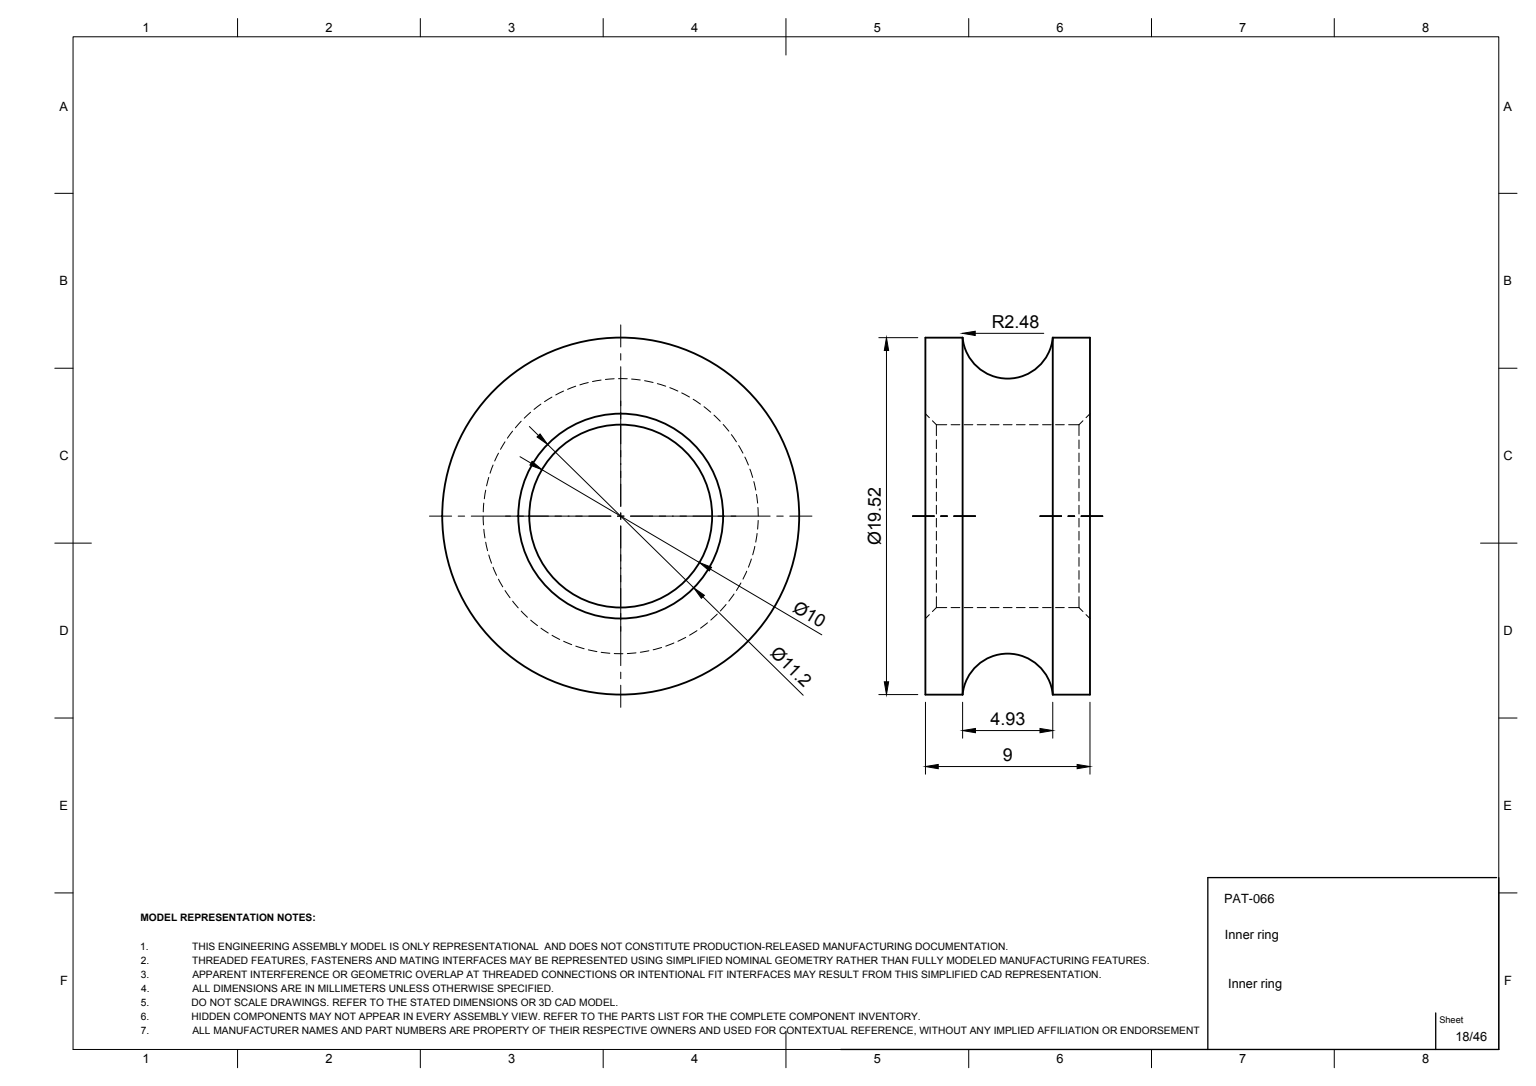
ISO-10303-21;
HEADER;
/* Generated by software containing ST-Developer
 * from STEP Tools, Inc. (www.steptools.com) 
 */

FILE_DESCRIPTION(
/* description */ ('Lever-operated bar clamp (toggle)'),
/* implementation_level */ '2;1');

FILE_NAME(
/* name */ 'Inner ring.step',
/* time_stamp */ '2026-10-28T03:25:02-07:00',
/* author */ (''),
/* organization */ (''),
/* preprocessor_version */ 'ST-DEVELOPER v20.2',
/* originating_system */ 'Autodesk Translation Framework v15.17.0.0',
/* authorisation */ '');

FILE_SCHEMA (('AUTOMOTIVE_DESIGN { 1 0 10303 214 3 1 1 }'));
ENDSEC;

DATA;
#10=MECHANICAL_DESIGN_GEOMETRIC_PRESENTATION_REPRESENTATION('',(#422),#12413);
#303=TOROIDAL_SURFACE('',#7329,1.,0.247676);
#308=CONICAL_SURFACE('',#7340,0.53,0.785398163397448);
#309=CONICAL_SURFACE('',#7347,0.53,0.785398163397448);
#346=SHAPE_REPRESENTATION_RELATIONSHIP('SRR','None',#12586,#384);
#384=ADVANCED_BREP_SHAPE_REPRESENTATION('',(#468),#12383);
#422=STYLED_ITEM('',(#12869),#468);
#468=MANIFOLD_SOLID_BREP('Body1',#6582);
#588=FACE_BOUND('',#1538,.T.);
#589=FACE_BOUND('',#1541,.T.);
#739=PLANE('',#7342);
#740=PLANE('',#7345);
#1039=FACE_OUTER_BOUND('',#1533,.T.);
#1040=FACE_OUTER_BOUND('',#1534,.T.);
#1041=FACE_OUTER_BOUND('',#1535,.T.);
#1042=FACE_OUTER_BOUND('',#1536,.T.);
#1043=FACE_OUTER_BOUND('',#1537,.T.);
#1044=FACE_OUTER_BOUND('',#1539,.T.);
#1045=FACE_OUTER_BOUND('',#1540,.T.);
#1046=FACE_OUTER_BOUND('',#1542,.T.);
#1533=EDGE_LOOP('',(#5045,#5046,#5047,#5048,#5049,#5050));
#1534=EDGE_LOOP('',(#5051,#5052,#5053,#5054,#5055));
#1535=EDGE_LOOP('',(#5056,#5057,#5058,#5059));
#1536=EDGE_LOOP('',(#5060,#5061,#5062,#5063));
#1537=EDGE_LOOP('',(#5064));
#1538=EDGE_LOOP('',(#5065));
#1539=EDGE_LOOP('',(#5066,#5067,#5068,#5069,#5070));
#1540=EDGE_LOOP('',(#5071));
#1541=EDGE_LOOP('',(#5072));
#1542=EDGE_LOOP('',(#5073,#5074,#5075,#5076));
#2040=LINE('',#10743,#2481);
#2041=LINE('',#10749,#2482);
#2042=LINE('',#10753,#2483);
#2043=LINE('',#10759,#2484);
#2044=LINE('',#10764,#2485);
#2481=VECTOR('',#8677,0.976185);
#2482=VECTOR('',#8684,0.5);
#2483=VECTOR('',#8689,0.53);
#2484=VECTOR('',#8698,0.976185);
#2485=VECTOR('',#8705,0.53);
#2856=CIRCLE('',#7330,0.976185);
#2857=CIRCLE('',#7331,0.976185);
#2858=CIRCLE('',#7332,0.247676);
#2859=CIRCLE('',#7333,0.976185);
#2860=CIRCLE('',#7334,0.976185);
#2861=CIRCLE('',#7336,0.976185);
#2862=CIRCLE('',#7338,0.5);
#2863=CIRCLE('',#7339,0.5);
#2864=CIRCLE('',#7341,0.56);
#2865=CIRCLE('',#7344,0.976185);
#2866=CIRCLE('',#7346,0.56);
#3281=VERTEX_POINT('',#10732);
#3282=VERTEX_POINT('',#10733);
#3283=VERTEX_POINT('',#10736);
#3284=VERTEX_POINT('',#10738);
#3285=VERTEX_POINT('',#10742);
#3286=VERTEX_POINT('',#10746);
#3287=VERTEX_POINT('',#10748);
#3288=VERTEX_POINT('',#10752);
#3289=VERTEX_POINT('',#10757);
#3290=VERTEX_POINT('',#10761);
#3927=EDGE_CURVE('',#3281,#3282,#2856,.T.);
#3928=EDGE_CURVE('',#3282,#3281,#2857,.T.);
#3929=EDGE_CURVE('',#3282,#3283,#2858,.T.);
#3930=EDGE_CURVE('',#3284,#3283,#2859,.T.);
#3931=EDGE_CURVE('',#3283,#3284,#2860,.T.);
#3932=EDGE_CURVE('',#3284,#3285,#2040,.T.);
#3933=EDGE_CURVE('',#3285,#3285,#2861,.T.);
#3934=EDGE_CURVE('',#3286,#3286,#2862,.T.);
#3935=EDGE_CURVE('',#3286,#3287,#2041,.T.);
#3936=EDGE_CURVE('',#3287,#3287,#2863,.T.);
#3937=EDGE_CURVE('',#3287,#3288,#2042,.T.);
#3938=EDGE_CURVE('',#3288,#3288,#2864,.T.);
#3939=EDGE_CURVE('',#3289,#3289,#2865,.T.);
#3940=EDGE_CURVE('',#3289,#3281,#2043,.T.);
#3941=EDGE_CURVE('',#3290,#3290,#2866,.T.);
#3942=EDGE_CURVE('',#3290,#3286,#2044,.T.);
#5045=ORIENTED_EDGE('',*,*,#3927,.F.);
#5046=ORIENTED_EDGE('',*,*,#3928,.F.);
#5047=ORIENTED_EDGE('',*,*,#3929,.T.);
#5048=ORIENTED_EDGE('',*,*,#3930,.F.);
#5049=ORIENTED_EDGE('',*,*,#3931,.F.);
#5050=ORIENTED_EDGE('',*,*,#3929,.F.);
#5051=ORIENTED_EDGE('',*,*,#3930,.T.);
#5052=ORIENTED_EDGE('',*,*,#3931,.T.);
#5053=ORIENTED_EDGE('',*,*,#3932,.T.);
#5054=ORIENTED_EDGE('',*,*,#3933,.T.);
#5055=ORIENTED_EDGE('',*,*,#3932,.F.);
#5056=ORIENTED_EDGE('',*,*,#3934,.T.);
#5057=ORIENTED_EDGE('',*,*,#3935,.T.);
#5058=ORIENTED_EDGE('',*,*,#3936,.F.);
#5059=ORIENTED_EDGE('',*,*,#3935,.F.);
#5060=ORIENTED_EDGE('',*,*,#3936,.T.);
#5061=ORIENTED_EDGE('',*,*,#3937,.T.);
#5062=ORIENTED_EDGE('',*,*,#3938,.F.);
#5063=ORIENTED_EDGE('',*,*,#3937,.F.);
#5064=ORIENTED_EDGE('',*,*,#3933,.F.);
#5065=ORIENTED_EDGE('',*,*,#3938,.T.);
#5066=ORIENTED_EDGE('',*,*,#3939,.F.);
#5067=ORIENTED_EDGE('',*,*,#3940,.T.);
#5068=ORIENTED_EDGE('',*,*,#3927,.T.);
#5069=ORIENTED_EDGE('',*,*,#3928,.T.);
#5070=ORIENTED_EDGE('',*,*,#3940,.F.);
#5071=ORIENTED_EDGE('',*,*,#3939,.T.);
#5072=ORIENTED_EDGE('',*,*,#3941,.F.);
#5073=ORIENTED_EDGE('',*,*,#3941,.T.);
#5074=ORIENTED_EDGE('',*,*,#3942,.T.);
#5075=ORIENTED_EDGE('',*,*,#3934,.F.);
#5076=ORIENTED_EDGE('',*,*,#3942,.F.);
#6093=CYLINDRICAL_SURFACE('',#7335,0.976185);
#6094=CYLINDRICAL_SURFACE('',#7337,0.5);
#6095=CYLINDRICAL_SURFACE('',#7343,0.976185);
#6314=ADVANCED_FACE('',(#1039),#303,.F.);
#6315=ADVANCED_FACE('',(#1040),#6093,.T.);
#6316=ADVANCED_FACE('',(#1041),#6094,.F.);
#6317=ADVANCED_FACE('',(#1042),#308,.F.);
#6318=ADVANCED_FACE('',(#1043,#588),#739,.T.);
#6319=ADVANCED_FACE('',(#1044),#6095,.T.);
#6320=ADVANCED_FACE('',(#1045,#589),#740,.T.);
#6321=ADVANCED_FACE('',(#1046),#309,.F.);
#6582=CLOSED_SHELL('',(#6314,#6315,#6316,#6317,#6318,#6319,#6320,#6321));
#7328=AXIS2_PLACEMENT_3D('',#10730,#8661,#8662);
#7329=AXIS2_PLACEMENT_3D('',#10731,#8663,#8664);
#7330=AXIS2_PLACEMENT_3D('',#10734,#8665,#8666);
#7331=AXIS2_PLACEMENT_3D('',#10735,#8667,#8668);
#7332=AXIS2_PLACEMENT_3D('',#10737,#8669,#8670);
#7333=AXIS2_PLACEMENT_3D('',#10739,#8671,#8672);
#7334=AXIS2_PLACEMENT_3D('',#10740,#8673,#8674);
#7335=AXIS2_PLACEMENT_3D('',#10741,#8675,#8676);
#7336=AXIS2_PLACEMENT_3D('',#10744,#8678,#8679);
#7337=AXIS2_PLACEMENT_3D('',#10745,#8680,#8681);
#7338=AXIS2_PLACEMENT_3D('',#10747,#8682,#8683);
#7339=AXIS2_PLACEMENT_3D('',#10750,#8685,#8686);
#7340=AXIS2_PLACEMENT_3D('',#10751,#8687,#8688);
#7341=AXIS2_PLACEMENT_3D('',#10754,#8690,#8691);
#7342=AXIS2_PLACEMENT_3D('',#10755,#8692,#8693);
#7343=AXIS2_PLACEMENT_3D('',#10756,#8694,#8695);
#7344=AXIS2_PLACEMENT_3D('',#10758,#8696,#8697);
#7345=AXIS2_PLACEMENT_3D('',#10760,#8699,#8700);
#7346=AXIS2_PLACEMENT_3D('',#10762,#8701,#8702);
#7347=AXIS2_PLACEMENT_3D('',#10763,#8703,#8704);
#8661=DIRECTION('axis',(0.,0.,1.));
#8662=DIRECTION('refdir',(1.,0.,0.));
#8663=DIRECTION('center_axis',(0.,-1.,0.));
#8664=DIRECTION('ref_axis',(0.,0.,-1.));
#8665=DIRECTION('center_axis',(0.,-1.,0.));
#8666=DIRECTION('ref_axis',(1.,0.,0.));
#8667=DIRECTION('center_axis',(0.,-1.,0.));
#8668=DIRECTION('ref_axis',(1.,0.,0.));
#8669=DIRECTION('center_axis',(1.,0.,1.22464679914735E-16));
#8670=DIRECTION('ref_axis',(-1.22464679914735E-16,0.,1.));
#8671=DIRECTION('center_axis',(0.,1.,0.));
#8672=DIRECTION('ref_axis',(1.,0.,0.));
#8673=DIRECTION('center_axis',(0.,1.,0.));
#8674=DIRECTION('ref_axis',(1.,0.,0.));
#8675=DIRECTION('center_axis',(0.,-1.,0.));
#8676=DIRECTION('ref_axis',(1.,0.,0.));
#8677=DIRECTION('',(0.,1.,0.));
#8678=DIRECTION('center_axis',(0.,-1.,0.));
#8679=DIRECTION('ref_axis',(1.,0.,0.));
#8680=DIRECTION('center_axis',(0.,-1.,0.));
#8681=DIRECTION('ref_axis',(1.,0.,0.));
#8682=DIRECTION('center_axis',(0.,-1.,0.));
#8683=DIRECTION('ref_axis',(1.,0.,0.));
#8684=DIRECTION('',(0.,1.,0.));
#8685=DIRECTION('center_axis',(0.,-1.,0.));
#8686=DIRECTION('ref_axis',(1.,0.,0.));
#8687=DIRECTION('center_axis',(0.,1.,0.));
#8688=DIRECTION('ref_axis',(1.,0.,0.));
#8689=DIRECTION('',(-0.707106781186547,0.707106781186548,-8.65956056235493E-17));
#8690=DIRECTION('center_axis',(0.,-1.,0.));
#8691=DIRECTION('ref_axis',(1.,0.,0.));
#8692=DIRECTION('center_axis',(0.,1.,0.));
#8693=DIRECTION('ref_axis',(0.,0.,1.));
#8694=DIRECTION('center_axis',(0.,-1.,0.));
#8695=DIRECTION('ref_axis',(1.,0.,0.));
#8696=DIRECTION('center_axis',(0.,-1.,0.));
#8697=DIRECTION('ref_axis',(1.,0.,0.));
#8698=DIRECTION('',(0.,1.,0.));
#8699=DIRECTION('center_axis',(0.,-1.,0.));
#8700=DIRECTION('ref_axis',(0.,0.,-1.));
#8701=DIRECTION('center_axis',(0.,-1.,0.));
#8702=DIRECTION('ref_axis',(1.,0.,0.));
#8703=DIRECTION('center_axis',(0.,-1.,0.));
#8704=DIRECTION('ref_axis',(1.,0.,0.));
#8705=DIRECTION('',(0.707106781186547,0.707106781186548,8.65956056235493E-17));
#10730=CARTESIAN_POINT('',(0.,0.,0.));
#10731=CARTESIAN_POINT('Origin',(0.,0.,0.));
#10732=CARTESIAN_POINT('',(-0.976185,-0.246528389340863,-1.19548183562566E-16));
#10733=CARTESIAN_POINT('',(-1.19548183562566E-16,-0.246528389340863,0.976185));
#10734=CARTESIAN_POINT('Origin',(0.,-0.246528389340863,0.));
#10735=CARTESIAN_POINT('Origin',(0.,-0.246528389340863,0.));
#10736=CARTESIAN_POINT('',(-1.19548183562566E-16,0.246528389340863,0.976185));
#10737=CARTESIAN_POINT('Origin',(-1.22464679914735E-16,0.,1.));
#10738=CARTESIAN_POINT('',(-0.976185,0.246528389340863,1.19548183562566E-16));
#10739=CARTESIAN_POINT('Origin',(0.,0.246528389340863,0.));
#10740=CARTESIAN_POINT('Origin',(0.,0.246528389340863,0.));
#10741=CARTESIAN_POINT('Origin',(0.,0.,0.));
#10742=CARTESIAN_POINT('',(-0.976185,0.45,-1.19548183562566E-16));
#10743=CARTESIAN_POINT('',(-0.976185,0.,-1.19548183562566E-16));
#10744=CARTESIAN_POINT('Origin',(0.,0.45,0.));
#10745=CARTESIAN_POINT('Origin',(0.,0.,0.));
#10746=CARTESIAN_POINT('',(-0.5,-0.39,-6.12323399573677E-17));
#10747=CARTESIAN_POINT('Origin',(0.,-0.39,0.));
#10748=CARTESIAN_POINT('',(-0.5,0.39,-6.12323399573677E-17));
#10749=CARTESIAN_POINT('',(-0.5,0.,-6.12323399573677E-17));
#10750=CARTESIAN_POINT('Origin',(0.,0.39,0.));
#10751=CARTESIAN_POINT('Origin',(0.,0.42,0.));
#10752=CARTESIAN_POINT('',(-0.56,0.45,-6.85802207522518E-17));
#10753=CARTESIAN_POINT('',(-0.53,0.42,-6.49062803548097E-17));
#10754=CARTESIAN_POINT('Origin',(0.,0.45,0.));
#10755=CARTESIAN_POINT('Origin',(0.976185,0.45,0.));
#10756=CARTESIAN_POINT('Origin',(0.,0.,0.));
#10757=CARTESIAN_POINT('',(-0.976185,-0.45,-1.19548183562566E-16));
#10758=CARTESIAN_POINT('Origin',(0.,-0.45,0.));
#10759=CARTESIAN_POINT('',(-0.976185,0.,-1.19548183562566E-16));
#10760=CARTESIAN_POINT('Origin',(0.56,-0.45,0.));
#10761=CARTESIAN_POINT('',(-0.56,-0.45,-6.85802207522518E-17));
#10762=CARTESIAN_POINT('Origin',(0.,-0.45,0.));
#10763=CARTESIAN_POINT('Origin',(0.,-0.42,0.));
#10764=CARTESIAN_POINT('',(-0.53,-0.42,-6.49062803548097E-17));
#12337=UNCERTAINTY_MEASURE_WITH_UNIT(LENGTH_MEASURE(0.001),#12414,
'DISTANCE_ACCURACY_VALUE',
'Maximum model space distance between geometric entities at asserted c
onnectivities');
#12367=UNCERTAINTY_MEASURE_WITH_UNIT(LENGTH_MEASURE(0.001),#12414,
'DISTANCE_ACCURACY_VALUE',
'Maximum model space distance between geometric entities at asserted c
onnectivities');
#12383=(
GEOMETRIC_REPRESENTATION_CONTEXT(3)
GLOBAL_UNCERTAINTY_ASSIGNED_CONTEXT((#12337))
GLOBAL_UNIT_ASSIGNED_CONTEXT((#12414,#12416,#12417))
REPRESENTATION_CONTEXT('','3D')
);
#12413=(
GEOMETRIC_REPRESENTATION_CONTEXT(3)
GLOBAL_UNCERTAINTY_ASSIGNED_CONTEXT((#12367))
GLOBAL_UNIT_ASSIGNED_CONTEXT((#12414,#12416,#12417))
REPRESENTATION_CONTEXT('','3D')
);
#12414=(
LENGTH_UNIT()
NAMED_UNIT(*)
SI_UNIT(.CENTI.,.METRE.)
);
#12416=(
NAMED_UNIT(*)
PLANE_ANGLE_UNIT()
SI_UNIT($,.RADIAN.)
);
#12417=(
NAMED_UNIT(*)
SI_UNIT($,.STERADIAN.)
SOLID_ANGLE_UNIT()
);
#12433=SHAPE_DEFINITION_REPRESENTATION(#12478,#12586);
#12478=PRODUCT_DEFINITION_SHAPE('',$,#12632);
#12586=SHAPE_REPRESENTATION('',(#7328),#12383);
#12616=PRODUCT_DEFINITION_CONTEXT('part definition',#12753,'design');
#12632=PRODUCT_DEFINITION('Inner ring','Inner ring',#12677,#12616);
#12677=PRODUCT_DEFINITION_FORMATION('',$,#12770);
#12753=APPLICATION_CONTEXT(
'Core Data for Automotive Mechanical Design Process');
#12754=PRODUCT_CONTEXT('part definition',#12753,'mechanical');
#12770=PRODUCT('Inner ring','Inner ring','Inner ring',(#12754));
#12863=COLOUR_RGB('Grey',0.48,0.52,0.57);
#12864=FILL_AREA_STYLE_COLOUR('',#12863);
#12865=FILL_AREA_STYLE('',(#12864));
#12866=SURFACE_STYLE_FILL_AREA(#12865);
#12867=SURFACE_SIDE_STYLE('',(#12866));
#12868=SURFACE_STYLE_USAGE(.BOTH.,#12867);
#12869=PRESENTATION_STYLE_ASSIGNMENT((#12868));
ENDSEC;
END-ISO-10303-21;
